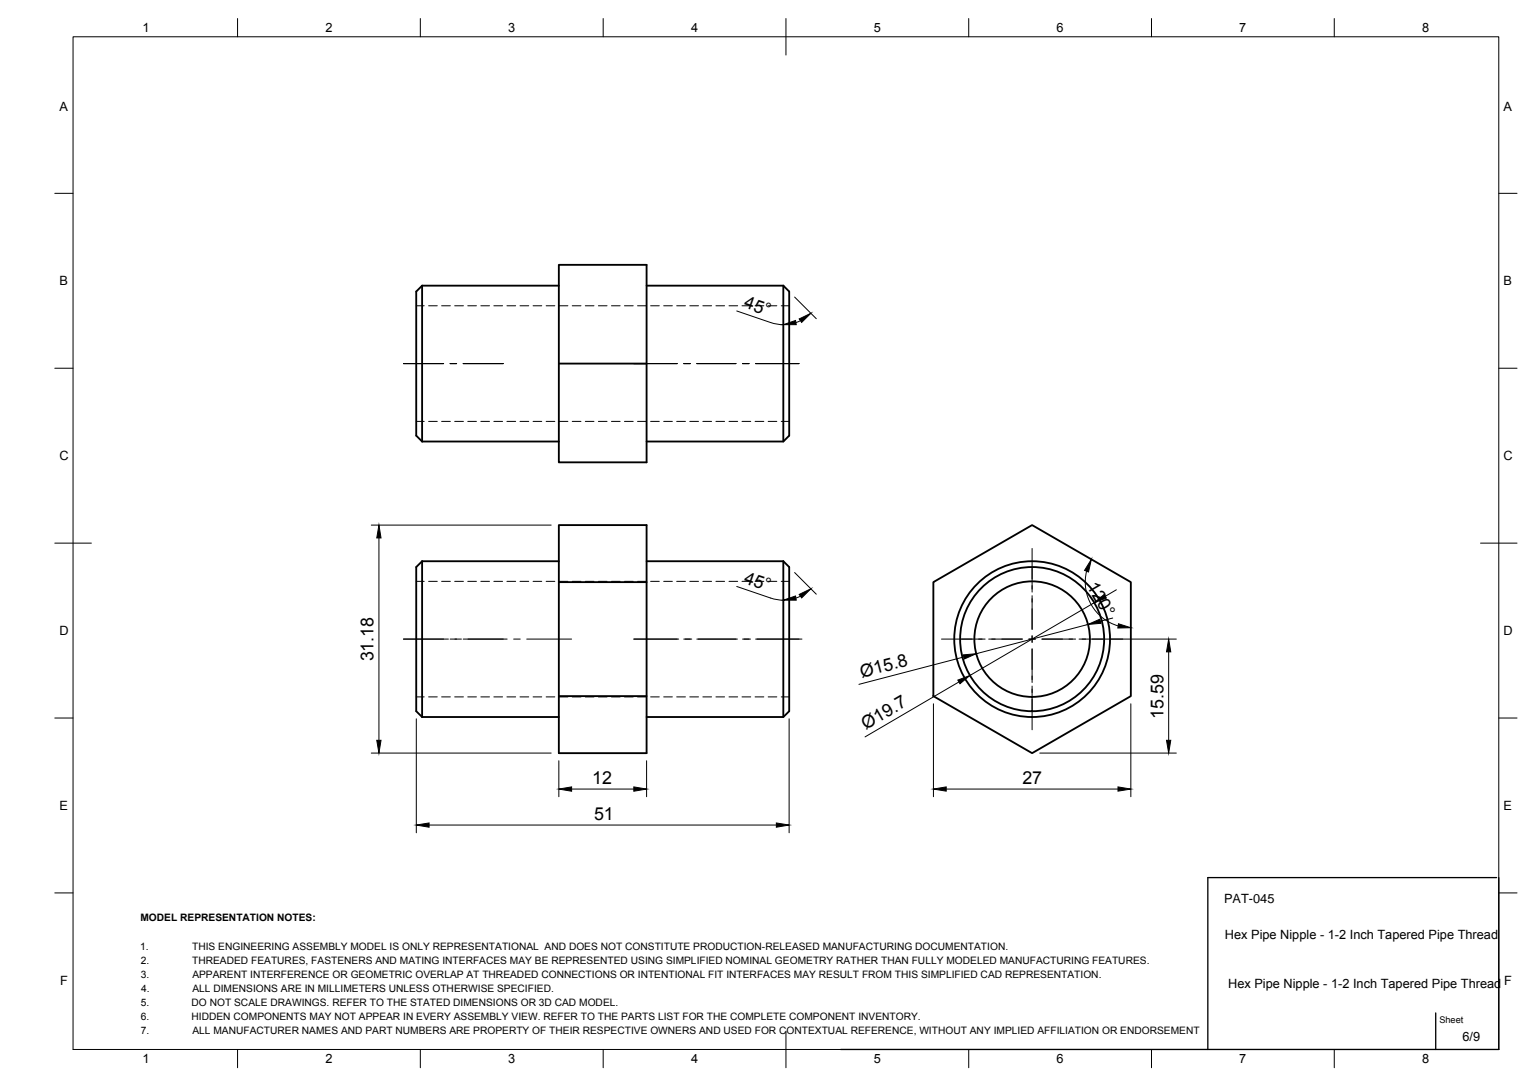
ISO-10303-21;
HEADER;
/* Generated by software containing ST-Developer
 * from STEP Tools, Inc. (www.steptools.com) 
 */

FILE_DESCRIPTION(
/* description */ ('Gauge isolation and snubber set'),
/* implementation_level */ '2;1');

FILE_NAME(
/* name */ 'Hex Pipe Nipple - 1-2 Inch Tapered Pipe Thread.step',
/* time_stamp */ '2026-10-29T16:58:15-07:00',
/* author */ (''),
/* organization */ (''),
/* preprocessor_version */ 'ST-DEVELOPER v20.2',
/* originating_system */ 'Autodesk Translation Framework v15.17.0.0',
/* authorisation */ '');

FILE_SCHEMA (('AUTOMOTIVE_DESIGN { 1 0 10303 214 3 1 1 }'));
ENDSEC;

DATA;
#10=MECHANICAL_DESIGN_GEOMETRIC_PRESENTATION_REPRESENTATION('',(#95),#4043);
#70=CONICAL_SURFACE('',#2483,1.025,0.785398163397448);
#71=CONICAL_SURFACE('',#2486,1.025,0.785398163397448);
#79=SHAPE_REPRESENTATION_RELATIONSHIP('SRR','None',#4086,#87);
#87=ADVANCED_BREP_SHAPE_REPRESENTATION('',(#105),#4038);
#95=STYLED_ITEM('',(#4183),#105);
#105=MANIFOLD_SOLID_BREP('Body1',#2212);
#146=FACE_BOUND('',#475,.T.);
#147=FACE_BOUND('',#477,.T.);
#148=FACE_BOUND('',#486,.T.);
#149=FACE_BOUND('',#491,.T.);
#208=PLANE('',#2468);
#209=PLANE('',#2470);
#210=PLANE('',#2472);
#211=PLANE('',#2473);
#212=PLANE('',#2474);
#213=PLANE('',#2475);
#214=PLANE('',#2476);
#215=PLANE('',#2477);
#216=PLANE('',#2480);
#217=PLANE('',#2488);
#316=FACE_OUTER_BOUND('',#474,.T.);
#317=FACE_OUTER_BOUND('',#476,.T.);
#318=FACE_OUTER_BOUND('',#478,.T.);
#319=FACE_OUTER_BOUND('',#479,.T.);
#320=FACE_OUTER_BOUND('',#480,.T.);
#321=FACE_OUTER_BOUND('',#481,.T.);
#322=FACE_OUTER_BOUND('',#482,.T.);
#323=FACE_OUTER_BOUND('',#483,.T.);
#324=FACE_OUTER_BOUND('',#484,.T.);
#325=FACE_OUTER_BOUND('',#485,.T.);
#326=FACE_OUTER_BOUND('',#487,.T.);
#327=FACE_OUTER_BOUND('',#488,.T.);
#328=FACE_OUTER_BOUND('',#489,.T.);
#329=FACE_OUTER_BOUND('',#490,.T.);
#330=FACE_OUTER_BOUND('',#492,.T.);
#474=EDGE_LOOP('',(#1863,#1864,#1865,#1866,#1867,#1868));
#475=EDGE_LOOP('',(#1869));
#476=EDGE_LOOP('',(#1870,#1871,#1872,#1873,#1874,#1875));
#477=EDGE_LOOP('',(#1876));
#478=EDGE_LOOP('',(#1877,#1878,#1879,#1880));
#479=EDGE_LOOP('',(#1881,#1882,#1883,#1884));
#480=EDGE_LOOP('',(#1885,#1886,#1887,#1888));
#481=EDGE_LOOP('',(#1889,#1890,#1891,#1892));
#482=EDGE_LOOP('',(#1893,#1894,#1895,#1896));
#483=EDGE_LOOP('',(#1897,#1898,#1899,#1900));
#484=EDGE_LOOP('',(#1901,#1902,#1903,#1904));
#485=EDGE_LOOP('',(#1905));
#486=EDGE_LOOP('',(#1906));
#487=EDGE_LOOP('',(#1907,#1908,#1909,#1910));
#488=EDGE_LOOP('',(#1911,#1912,#1913,#1914));
#489=EDGE_LOOP('',(#1915,#1916,#1917,#1918));
#490=EDGE_LOOP('',(#1919));
#491=EDGE_LOOP('',(#1920));
#492=EDGE_LOOP('',(#1921,#1922,#1923,#1924));
#609=CIRCLE('',#2469,1.065);
#610=CIRCLE('',#2471,1.065);
#611=CIRCLE('',#2479,1.065);
#612=CIRCLE('',#2481,0.985);
#613=CIRCLE('',#2482,0.79);
#614=CIRCLE('',#2485,1.065);
#615=CIRCLE('',#2487,0.985);
#616=CIRCLE('',#2489,0.79);
#745=LINE('',#3797,#916);
#746=LINE('',#3799,#917);
#747=LINE('',#3801,#918);
#748=LINE('',#3803,#919);
#749=LINE('',#3805,#920);
#750=LINE('',#3806,#921);
#751=LINE('',#3812,#922);
#752=LINE('',#3814,#923);
#753=LINE('',#3816,#924);
#754=LINE('',#3818,#925);
#755=LINE('',#3820,#926);
#756=LINE('',#3821,#927);
#757=LINE('',#3825,#928);
#758=LINE('',#3826,#929);
#759=LINE('',#3828,#930);
#760=LINE('',#3830,#931);
#761=LINE('',#3832,#932);
#762=LINE('',#3834,#933);
#763=LINE('',#3838,#934);
#764=LINE('',#3846,#935);
#765=LINE('',#3850,#936);
#766=LINE('',#3854,#937);
#767=LINE('',#3859,#938);
#916=VECTOR('',#2992,1.);
#917=VECTOR('',#2993,1.);
#918=VECTOR('',#2994,1.);
#919=VECTOR('',#2995,1.);
#920=VECTOR('',#2996,1.);
#921=VECTOR('',#2997,1.);
#922=VECTOR('',#3002,1.);
#923=VECTOR('',#3003,1.);
#924=VECTOR('',#3004,1.);
#925=VECTOR('',#3005,1.);
#926=VECTOR('',#3006,1.);
#927=VECTOR('',#3007,1.);
#928=VECTOR('',#3012,1.);
#929=VECTOR('',#3013,1.);
#930=VECTOR('',#3016,1.);
#931=VECTOR('',#3019,1.);
#932=VECTOR('',#3022,1.);
#933=VECTOR('',#3025,1.);
#934=VECTOR('',#3030,1.065);
#935=VECTOR('',#3041,1.025);
#936=VECTOR('',#3046,1.065);
#937=VECTOR('',#3051,1.025);
#938=VECTOR('',#3058,0.79);
#1110=VERTEX_POINT('',#3795);
#1111=VERTEX_POINT('',#3796);
#1112=VERTEX_POINT('',#3798);
#1113=VERTEX_POINT('',#3800);
#1114=VERTEX_POINT('',#3802);
#1115=VERTEX_POINT('',#3804);
#1116=VERTEX_POINT('',#3807);
#1117=VERTEX_POINT('',#3810);
#1118=VERTEX_POINT('',#3811);
#1119=VERTEX_POINT('',#3813);
#1120=VERTEX_POINT('',#3815);
#1121=VERTEX_POINT('',#3817);
#1122=VERTEX_POINT('',#3819);
#1123=VERTEX_POINT('',#3822);
#1124=VERTEX_POINT('',#3837);
#1125=VERTEX_POINT('',#3841);
#1126=VERTEX_POINT('',#3843);
#1127=VERTEX_POINT('',#3848);
#1128=VERTEX_POINT('',#3852);
#1129=VERTEX_POINT('',#3856);
#1370=EDGE_CURVE('',#1110,#1111,#745,.T.);
#1371=EDGE_CURVE('',#1111,#1112,#746,.T.);
#1372=EDGE_CURVE('',#1112,#1113,#747,.T.);
#1373=EDGE_CURVE('',#1113,#1114,#748,.T.);
#1374=EDGE_CURVE('',#1114,#1115,#749,.T.);
#1375=EDGE_CURVE('',#1115,#1110,#750,.T.);
#1376=EDGE_CURVE('',#1116,#1116,#609,.T.);
#1377=EDGE_CURVE('',#1117,#1118,#751,.T.);
#1378=EDGE_CURVE('',#1118,#1119,#752,.T.);
#1379=EDGE_CURVE('',#1119,#1120,#753,.T.);
#1380=EDGE_CURVE('',#1120,#1121,#754,.T.);
#1381=EDGE_CURVE('',#1121,#1122,#755,.T.);
#1382=EDGE_CURVE('',#1122,#1117,#756,.T.);
#1383=EDGE_CURVE('',#1123,#1123,#610,.T.);
#1384=EDGE_CURVE('',#1117,#1111,#757,.T.);
#1385=EDGE_CURVE('',#1112,#1122,#758,.T.);
#1386=EDGE_CURVE('',#1113,#1121,#759,.T.);
#1387=EDGE_CURVE('',#1114,#1120,#760,.T.);
#1388=EDGE_CURVE('',#1115,#1119,#761,.T.);
#1389=EDGE_CURVE('',#1110,#1118,#762,.T.);
#1390=EDGE_CURVE('',#1123,#1124,#763,.T.);
#1391=EDGE_CURVE('',#1124,#1124,#611,.T.);
#1392=EDGE_CURVE('',#1125,#1125,#612,.T.);
#1393=EDGE_CURVE('',#1126,#1126,#613,.T.);
#1394=EDGE_CURVE('',#1124,#1125,#764,.T.);
#1395=EDGE_CURVE('',#1127,#1127,#614,.T.);
#1396=EDGE_CURVE('',#1127,#1116,#765,.T.);
#1397=EDGE_CURVE('',#1128,#1128,#615,.T.);
#1398=EDGE_CURVE('',#1128,#1127,#766,.T.);
#1399=EDGE_CURVE('',#1129,#1129,#616,.T.);
#1400=EDGE_CURVE('',#1129,#1126,#767,.T.);
#1863=ORIENTED_EDGE('',*,*,#1370,.T.);
#1864=ORIENTED_EDGE('',*,*,#1371,.T.);
#1865=ORIENTED_EDGE('',*,*,#1372,.T.);
#1866=ORIENTED_EDGE('',*,*,#1373,.T.);
#1867=ORIENTED_EDGE('',*,*,#1374,.T.);
#1868=ORIENTED_EDGE('',*,*,#1375,.T.);
#1869=ORIENTED_EDGE('',*,*,#1376,.F.);
#1870=ORIENTED_EDGE('',*,*,#1377,.T.);
#1871=ORIENTED_EDGE('',*,*,#1378,.T.);
#1872=ORIENTED_EDGE('',*,*,#1379,.T.);
#1873=ORIENTED_EDGE('',*,*,#1380,.T.);
#1874=ORIENTED_EDGE('',*,*,#1381,.T.);
#1875=ORIENTED_EDGE('',*,*,#1382,.T.);
#1876=ORIENTED_EDGE('',*,*,#1383,.F.);
#1877=ORIENTED_EDGE('',*,*,#1384,.F.);
#1878=ORIENTED_EDGE('',*,*,#1382,.F.);
#1879=ORIENTED_EDGE('',*,*,#1385,.F.);
#1880=ORIENTED_EDGE('',*,*,#1371,.F.);
#1881=ORIENTED_EDGE('',*,*,#1385,.T.);
#1882=ORIENTED_EDGE('',*,*,#1381,.F.);
#1883=ORIENTED_EDGE('',*,*,#1386,.F.);
#1884=ORIENTED_EDGE('',*,*,#1372,.F.);
#1885=ORIENTED_EDGE('',*,*,#1386,.T.);
#1886=ORIENTED_EDGE('',*,*,#1380,.F.);
#1887=ORIENTED_EDGE('',*,*,#1387,.F.);
#1888=ORIENTED_EDGE('',*,*,#1373,.F.);
#1889=ORIENTED_EDGE('',*,*,#1387,.T.);
#1890=ORIENTED_EDGE('',*,*,#1379,.F.);
#1891=ORIENTED_EDGE('',*,*,#1388,.F.);
#1892=ORIENTED_EDGE('',*,*,#1374,.F.);
#1893=ORIENTED_EDGE('',*,*,#1388,.T.);
#1894=ORIENTED_EDGE('',*,*,#1378,.F.);
#1895=ORIENTED_EDGE('',*,*,#1389,.F.);
#1896=ORIENTED_EDGE('',*,*,#1375,.F.);
#1897=ORIENTED_EDGE('',*,*,#1389,.T.);
#1898=ORIENTED_EDGE('',*,*,#1377,.F.);
#1899=ORIENTED_EDGE('',*,*,#1384,.T.);
#1900=ORIENTED_EDGE('',*,*,#1370,.F.);
#1901=ORIENTED_EDGE('',*,*,#1383,.T.);
#1902=ORIENTED_EDGE('',*,*,#1390,.T.);
#1903=ORIENTED_EDGE('',*,*,#1391,.T.);
#1904=ORIENTED_EDGE('',*,*,#1390,.F.);
#1905=ORIENTED_EDGE('',*,*,#1392,.F.);
#1906=ORIENTED_EDGE('',*,*,#1393,.T.);
#1907=ORIENTED_EDGE('',*,*,#1391,.F.);
#1908=ORIENTED_EDGE('',*,*,#1394,.T.);
#1909=ORIENTED_EDGE('',*,*,#1392,.T.);
#1910=ORIENTED_EDGE('',*,*,#1394,.F.);
#1911=ORIENTED_EDGE('',*,*,#1395,.F.);
#1912=ORIENTED_EDGE('',*,*,#1396,.T.);
#1913=ORIENTED_EDGE('',*,*,#1376,.T.);
#1914=ORIENTED_EDGE('',*,*,#1396,.F.);
#1915=ORIENTED_EDGE('',*,*,#1397,.F.);
#1916=ORIENTED_EDGE('',*,*,#1398,.T.);
#1917=ORIENTED_EDGE('',*,*,#1395,.T.);
#1918=ORIENTED_EDGE('',*,*,#1398,.F.);
#1919=ORIENTED_EDGE('',*,*,#1397,.T.);
#1920=ORIENTED_EDGE('',*,*,#1399,.F.);
#1921=ORIENTED_EDGE('',*,*,#1399,.T.);
#1922=ORIENTED_EDGE('',*,*,#1400,.T.);
#1923=ORIENTED_EDGE('',*,*,#1393,.F.);
#1924=ORIENTED_EDGE('',*,*,#1400,.F.);
#2076=CYLINDRICAL_SURFACE('',#2478,1.065);
#2077=CYLINDRICAL_SURFACE('',#2484,1.065);
#2078=CYLINDRICAL_SURFACE('',#2490,0.79);
#2160=ADVANCED_FACE('',(#316,#146),#208,.F.);
#2161=ADVANCED_FACE('',(#317,#147),#209,.T.);
#2162=ADVANCED_FACE('',(#318),#210,.T.);
#2163=ADVANCED_FACE('',(#319),#211,.T.);
#2164=ADVANCED_FACE('',(#320),#212,.T.);
#2165=ADVANCED_FACE('',(#321),#213,.T.);
#2166=ADVANCED_FACE('',(#322),#214,.T.);
#2167=ADVANCED_FACE('',(#323),#215,.T.);
#2168=ADVANCED_FACE('',(#324),#2076,.T.);
#2169=ADVANCED_FACE('',(#325,#148),#216,.T.);
#2170=ADVANCED_FACE('',(#326),#70,.T.);
#2171=ADVANCED_FACE('',(#327),#2077,.T.);
#2172=ADVANCED_FACE('',(#328),#71,.T.);
#2173=ADVANCED_FACE('',(#329,#149),#217,.T.);
#2174=ADVANCED_FACE('',(#330),#2078,.F.);
#2212=CLOSED_SHELL('',(#2160,#2161,#2162,#2163,#2164,#2165,#2166,#2167,
#2168,#2169,#2170,#2171,#2172,#2173,#2174));
#2467=AXIS2_PLACEMENT_3D('',#3793,#2988,#2989);
#2468=AXIS2_PLACEMENT_3D('',#3794,#2990,#2991);
#2469=AXIS2_PLACEMENT_3D('',#3808,#2998,#2999);
#2470=AXIS2_PLACEMENT_3D('',#3809,#3000,#3001);
#2471=AXIS2_PLACEMENT_3D('',#3823,#3008,#3009);
#2472=AXIS2_PLACEMENT_3D('',#3824,#3010,#3011);
#2473=AXIS2_PLACEMENT_3D('',#3827,#3014,#3015);
#2474=AXIS2_PLACEMENT_3D('',#3829,#3017,#3018);
#2475=AXIS2_PLACEMENT_3D('',#3831,#3020,#3021);
#2476=AXIS2_PLACEMENT_3D('',#3833,#3023,#3024);
#2477=AXIS2_PLACEMENT_3D('',#3835,#3026,#3027);
#2478=AXIS2_PLACEMENT_3D('',#3836,#3028,#3029);
#2479=AXIS2_PLACEMENT_3D('',#3839,#3031,#3032);
#2480=AXIS2_PLACEMENT_3D('',#3840,#3033,#3034);
#2481=AXIS2_PLACEMENT_3D('',#3842,#3035,#3036);
#2482=AXIS2_PLACEMENT_3D('',#3844,#3037,#3038);
#2483=AXIS2_PLACEMENT_3D('',#3845,#3039,#3040);
#2484=AXIS2_PLACEMENT_3D('',#3847,#3042,#3043);
#2485=AXIS2_PLACEMENT_3D('',#3849,#3044,#3045);
#2486=AXIS2_PLACEMENT_3D('',#3851,#3047,#3048);
#2487=AXIS2_PLACEMENT_3D('',#3853,#3049,#3050);
#2488=AXIS2_PLACEMENT_3D('',#3855,#3052,#3053);
#2489=AXIS2_PLACEMENT_3D('',#3857,#3054,#3055);
#2490=AXIS2_PLACEMENT_3D('',#3858,#3056,#3057);
#2988=DIRECTION('axis',(0.,0.,1.));
#2989=DIRECTION('refdir',(1.,0.,0.));
#2990=DIRECTION('center_axis',(0.,1.,0.));
#2991=DIRECTION('ref_axis',(1.,0.,0.));
#2992=DIRECTION('',(-0.5,0.,0.866025403784439));
#2993=DIRECTION('',(-1.,0.,-2.84883360945713E-16));
#2994=DIRECTION('',(-0.5,0.,-0.866025403784439));
#2995=DIRECTION('',(0.5,0.,-0.866025403784439));
#2996=DIRECTION('',(1.,0.,0.));
#2997=DIRECTION('',(0.5,0.,0.866025403784439));
#2998=DIRECTION('center_axis',(0.,-1.,0.));
#2999=DIRECTION('ref_axis',(1.,0.,0.));
#3000=DIRECTION('center_axis',(0.,1.,0.));
#3001=DIRECTION('ref_axis',(1.,0.,0.));
#3002=DIRECTION('',(0.5,0.,-0.866025403784439));
#3003=DIRECTION('',(-0.5,0.,-0.866025403784439));
#3004=DIRECTION('',(-1.,0.,0.));
#3005=DIRECTION('',(-0.5,0.,0.866025403784439));
#3006=DIRECTION('',(0.5,0.,0.866025403784439));
#3007=DIRECTION('',(1.,0.,2.84883360945713E-16));
#3008=DIRECTION('center_axis',(0.,1.,0.));
#3009=DIRECTION('ref_axis',(1.,0.,0.));
#3010=DIRECTION('center_axis',(-2.84883360945713E-16,0.,1.));
#3011=DIRECTION('ref_axis',(1.,0.,2.84883360945713E-16));
#3012=DIRECTION('',(0.,-1.,0.));
#3013=DIRECTION('',(0.,1.,0.));
#3014=DIRECTION('center_axis',(-0.866025403784439,0.,0.5));
#3015=DIRECTION('ref_axis',(0.5,0.,0.866025403784439));
#3016=DIRECTION('',(0.,1.,0.));
#3017=DIRECTION('center_axis',(-0.866025403784439,0.,-0.5));
#3018=DIRECTION('ref_axis',(-0.5,0.,0.866025403784439));
#3019=DIRECTION('',(0.,1.,0.));
#3020=DIRECTION('center_axis',(0.,0.,-1.));
#3021=DIRECTION('ref_axis',(-1.,0.,0.));
#3022=DIRECTION('',(0.,1.,0.));
#3023=DIRECTION('center_axis',(0.866025403784439,0.,-0.5));
#3024=DIRECTION('ref_axis',(-0.5,0.,-0.866025403784439));
#3025=DIRECTION('',(0.,1.,0.));
#3026=DIRECTION('center_axis',(0.866025403784439,0.,0.5));
#3027=DIRECTION('ref_axis',(0.5,0.,-0.866025403784439));
#3028=DIRECTION('center_axis',(0.,-1.,0.));
#3029=DIRECTION('ref_axis',(1.,0.,0.));
#3030=DIRECTION('',(0.,1.,0.));
#3031=DIRECTION('center_axis',(0.,-1.,0.));
#3032=DIRECTION('ref_axis',(1.,0.,0.));
#3033=DIRECTION('center_axis',(0.,1.,0.));
#3034=DIRECTION('ref_axis',(0.,0.,1.));
#3035=DIRECTION('center_axis',(0.,-1.,0.));
#3036=DIRECTION('ref_axis',(1.,0.,0.));
#3037=DIRECTION('center_axis',(0.,-1.,0.));
#3038=DIRECTION('ref_axis',(1.,0.,0.));
#3039=DIRECTION('center_axis',(0.,-1.,0.));
#3040=DIRECTION('ref_axis',(1.,0.,0.));
#3041=DIRECTION('',(0.707106781186547,0.707106781186548,8.65956056235493E-17));
#3042=DIRECTION('center_axis',(0.,-1.,0.));
#3043=DIRECTION('ref_axis',(1.,0.,0.));
#3044=DIRECTION('center_axis',(0.,-1.,0.));
#3045=DIRECTION('ref_axis',(1.,0.,0.));
#3046=DIRECTION('',(0.,1.,0.));
#3047=DIRECTION('center_axis',(0.,1.,0.));
#3048=DIRECTION('ref_axis',(1.,0.,0.));
#3049=DIRECTION('center_axis',(0.,-1.,0.));
#3050=DIRECTION('ref_axis',(1.,0.,0.));
#3051=DIRECTION('',(-0.707106781186547,0.707106781186548,-8.65956056235493E-17));
#3052=DIRECTION('center_axis',(0.,-1.,0.));
#3053=DIRECTION('ref_axis',(0.,0.,-1.));
#3054=DIRECTION('center_axis',(0.,-1.,0.));
#3055=DIRECTION('ref_axis',(1.,0.,0.));
#3056=DIRECTION('center_axis',(0.,-1.,0.));
#3057=DIRECTION('ref_axis',(1.,0.,0.));
#3058=DIRECTION('',(0.,1.,0.));
#3793=CARTESIAN_POINT('',(0.,0.,0.));
#3794=CARTESIAN_POINT('Origin',(0.,-0.6,0.));
#3795=CARTESIAN_POINT('',(1.55884572681199,-0.6,0.));
#3796=CARTESIAN_POINT('',(0.779422863405995,-0.6,1.35));
#3797=CARTESIAN_POINT('',(0.779422863405995,-0.6,1.35));
#3798=CARTESIAN_POINT('',(-0.779422863405996,-0.6,1.35));
#3799=CARTESIAN_POINT('',(-0.779422863405996,-0.6,1.35));
#3800=CARTESIAN_POINT('',(-1.55884572681199,-0.6,-1.90903542970483E-16));
#3801=CARTESIAN_POINT('',(-1.55884572681199,-0.6,-1.90903542970483E-16));
#3802=CARTESIAN_POINT('',(-0.779422863405995,-0.6,-1.35));
#3803=CARTESIAN_POINT('',(-0.779422863405995,-0.6,-1.35));
#3804=CARTESIAN_POINT('',(0.779422863405995,-0.6,-1.35));
#3805=CARTESIAN_POINT('',(0.779422863405995,-0.6,-1.35));
#3806=CARTESIAN_POINT('',(1.55884572681199,-0.6,0.));
#3807=CARTESIAN_POINT('',(-1.065,-0.6,-1.30424884109193E-16));
#3808=CARTESIAN_POINT('Origin',(0.,-0.6,0.));
#3809=CARTESIAN_POINT('Origin',(0.,0.6,0.));
#3810=CARTESIAN_POINT('',(0.779422863405995,0.6,1.35));
#3811=CARTESIAN_POINT('',(1.55884572681199,0.6,0.));
#3812=CARTESIAN_POINT('',(0.779422863405995,0.6,1.35));
#3813=CARTESIAN_POINT('',(0.779422863405995,0.6,-1.35));
#3814=CARTESIAN_POINT('',(1.55884572681199,0.6,0.));
#3815=CARTESIAN_POINT('',(-0.779422863405995,0.6,-1.35));
#3816=CARTESIAN_POINT('',(0.779422863405995,0.6,-1.35));
#3817=CARTESIAN_POINT('',(-1.55884572681199,0.6,-1.90903542970483E-16));
#3818=CARTESIAN_POINT('',(-0.779422863405995,0.6,-1.35));
#3819=CARTESIAN_POINT('',(-0.779422863405996,0.6,1.35));
#3820=CARTESIAN_POINT('',(-1.55884572681199,0.6,-1.90903542970483E-16));
#3821=CARTESIAN_POINT('',(-0.779422863405996,0.6,1.35));
#3822=CARTESIAN_POINT('',(-1.065,0.6,1.30424884109193E-16));
#3823=CARTESIAN_POINT('Origin',(0.,0.6,0.));
#3824=CARTESIAN_POINT('Origin',(-0.779422863405996,0.,1.35));
#3825=CARTESIAN_POINT('',(0.779422863405995,0.,1.35));
#3826=CARTESIAN_POINT('',(-0.779422863405996,0.,1.35));
#3827=CARTESIAN_POINT('Origin',(-1.55884572681199,0.,-1.90903542970483E-16));
#3828=CARTESIAN_POINT('',(-1.55884572681199,0.,-1.90903542970483E-16));
#3829=CARTESIAN_POINT('Origin',(-0.779422863405995,0.,-1.35));
#3830=CARTESIAN_POINT('',(-0.779422863405995,0.,-1.35));
#3831=CARTESIAN_POINT('Origin',(0.779422863405995,0.,-1.35));
#3832=CARTESIAN_POINT('',(0.779422863405995,0.,-1.35));
#3833=CARTESIAN_POINT('Origin',(1.55884572681199,0.,0.));
#3834=CARTESIAN_POINT('',(1.55884572681199,0.,0.));
#3835=CARTESIAN_POINT('Origin',(0.779422863405995,0.,1.35));
#3836=CARTESIAN_POINT('Origin',(0.,0.,0.));
#3837=CARTESIAN_POINT('',(-1.065,2.47,-1.30424884109193E-16));
#3838=CARTESIAN_POINT('',(-1.065,0.,-1.30424884109193E-16));
#3839=CARTESIAN_POINT('Origin',(0.,2.47,0.));
#3840=CARTESIAN_POINT('Origin',(0.985,2.55,0.));
#3841=CARTESIAN_POINT('',(-0.985,2.55,-1.20627709716014E-16));
#3842=CARTESIAN_POINT('Origin',(0.,2.55,0.));
#3843=CARTESIAN_POINT('',(-0.79,2.55,-9.67470971326409E-17));
#3844=CARTESIAN_POINT('Origin',(0.,2.55,0.));
#3845=CARTESIAN_POINT('Origin',(0.,2.51,0.));
#3846=CARTESIAN_POINT('',(-1.025,2.51,-1.25526296912604E-16));
#3847=CARTESIAN_POINT('Origin',(0.,0.,0.));
#3848=CARTESIAN_POINT('',(-1.065,-2.47,-1.30424884109193E-16));
#3849=CARTESIAN_POINT('Origin',(0.,-2.47,0.));
#3850=CARTESIAN_POINT('',(-1.065,0.,-1.30424884109193E-16));
#3851=CARTESIAN_POINT('Origin',(0.,-2.51,0.));
#3852=CARTESIAN_POINT('',(-0.985,-2.55,-1.20627709716014E-16));
#3853=CARTESIAN_POINT('Origin',(0.,-2.55,0.));
#3854=CARTESIAN_POINT('',(-1.025,-2.51,-1.25526296912604E-16));
#3855=CARTESIAN_POINT('Origin',(0.79,-2.55,0.));
#3856=CARTESIAN_POINT('',(-0.79,-2.55,-9.67470971326409E-17));
#3857=CARTESIAN_POINT('Origin',(0.,-2.55,0.));
#3858=CARTESIAN_POINT('Origin',(0.,0.,0.));
#3859=CARTESIAN_POINT('',(-0.79,0.,-9.67470971326409E-17));
#4027=UNCERTAINTY_MEASURE_WITH_UNIT(LENGTH_MEASURE(0.001),#4044,
'DISTANCE_ACCURACY_VALUE',
'Maximum model space distance between geometric entities at asserted c
onnectivities');
#4032=UNCERTAINTY_MEASURE_WITH_UNIT(LENGTH_MEASURE(0.001),#4044,
'DISTANCE_ACCURACY_VALUE',
'Maximum model space distance between geometric entities at asserted c
onnectivities');
#4038=(
GEOMETRIC_REPRESENTATION_CONTEXT(3)
GLOBAL_UNCERTAINTY_ASSIGNED_CONTEXT((#4027))
GLOBAL_UNIT_ASSIGNED_CONTEXT((#4044,#4046,#4047))
REPRESENTATION_CONTEXT('','3D')
);
#4043=(
GEOMETRIC_REPRESENTATION_CONTEXT(3)
GLOBAL_UNCERTAINTY_ASSIGNED_CONTEXT((#4032))
GLOBAL_UNIT_ASSIGNED_CONTEXT((#4044,#4046,#4047))
REPRESENTATION_CONTEXT('','3D')
);
#4044=(
LENGTH_UNIT()
NAMED_UNIT(*)
SI_UNIT(.CENTI.,.METRE.)
);
#4046=(
NAMED_UNIT(*)
PLANE_ANGLE_UNIT()
SI_UNIT($,.RADIAN.)
);
#4047=(
NAMED_UNIT(*)
SI_UNIT($,.STERADIAN.)
SOLID_ANGLE_UNIT()
);
#4053=SHAPE_DEFINITION_REPRESENTATION(#4063,#4086);
#4063=PRODUCT_DEFINITION_SHAPE('',$,#4097);
#4086=SHAPE_REPRESENTATION('',(#2467),#4038);
#4091=PRODUCT_DEFINITION_CONTEXT('part definition',#4123,'design');
#4097=PRODUCT_DEFINITION(
'Hex Pipe Nipple - 1-2 Inch Tapered Pipe Thread',
'Hex Pipe Nipple - 1-2 Inch Tapered Pipe Thread',#4107,#4091);
#4107=PRODUCT_DEFINITION_FORMATION('',$,#4130);
#4123=APPLICATION_CONTEXT(
'Core Data for Automotive Mechanical Design Process');
#4124=PRODUCT_CONTEXT('part definition',#4123,'mechanical');
#4130=PRODUCT('Hex Pipe Nipple - 1-2 Inch Tapered Pipe Thread',
'Hex Pipe Nipple - 1-2 Inch Tapered Pipe Thread',
'Hex Pipe Nipple - 1-2 Inch Tapered Pipe Thread',(#4124));
#4177=COLOUR_RGB('Light Blue',0.38,0.62,0.78);
#4178=FILL_AREA_STYLE_COLOUR('',#4177);
#4179=FILL_AREA_STYLE('',(#4178));
#4180=SURFACE_STYLE_FILL_AREA(#4179);
#4181=SURFACE_SIDE_STYLE('',(#4180));
#4182=SURFACE_STYLE_USAGE(.BOTH.,#4181);
#4183=PRESENTATION_STYLE_ASSIGNMENT((#4182));
ENDSEC;
END-ISO-10303-21;
